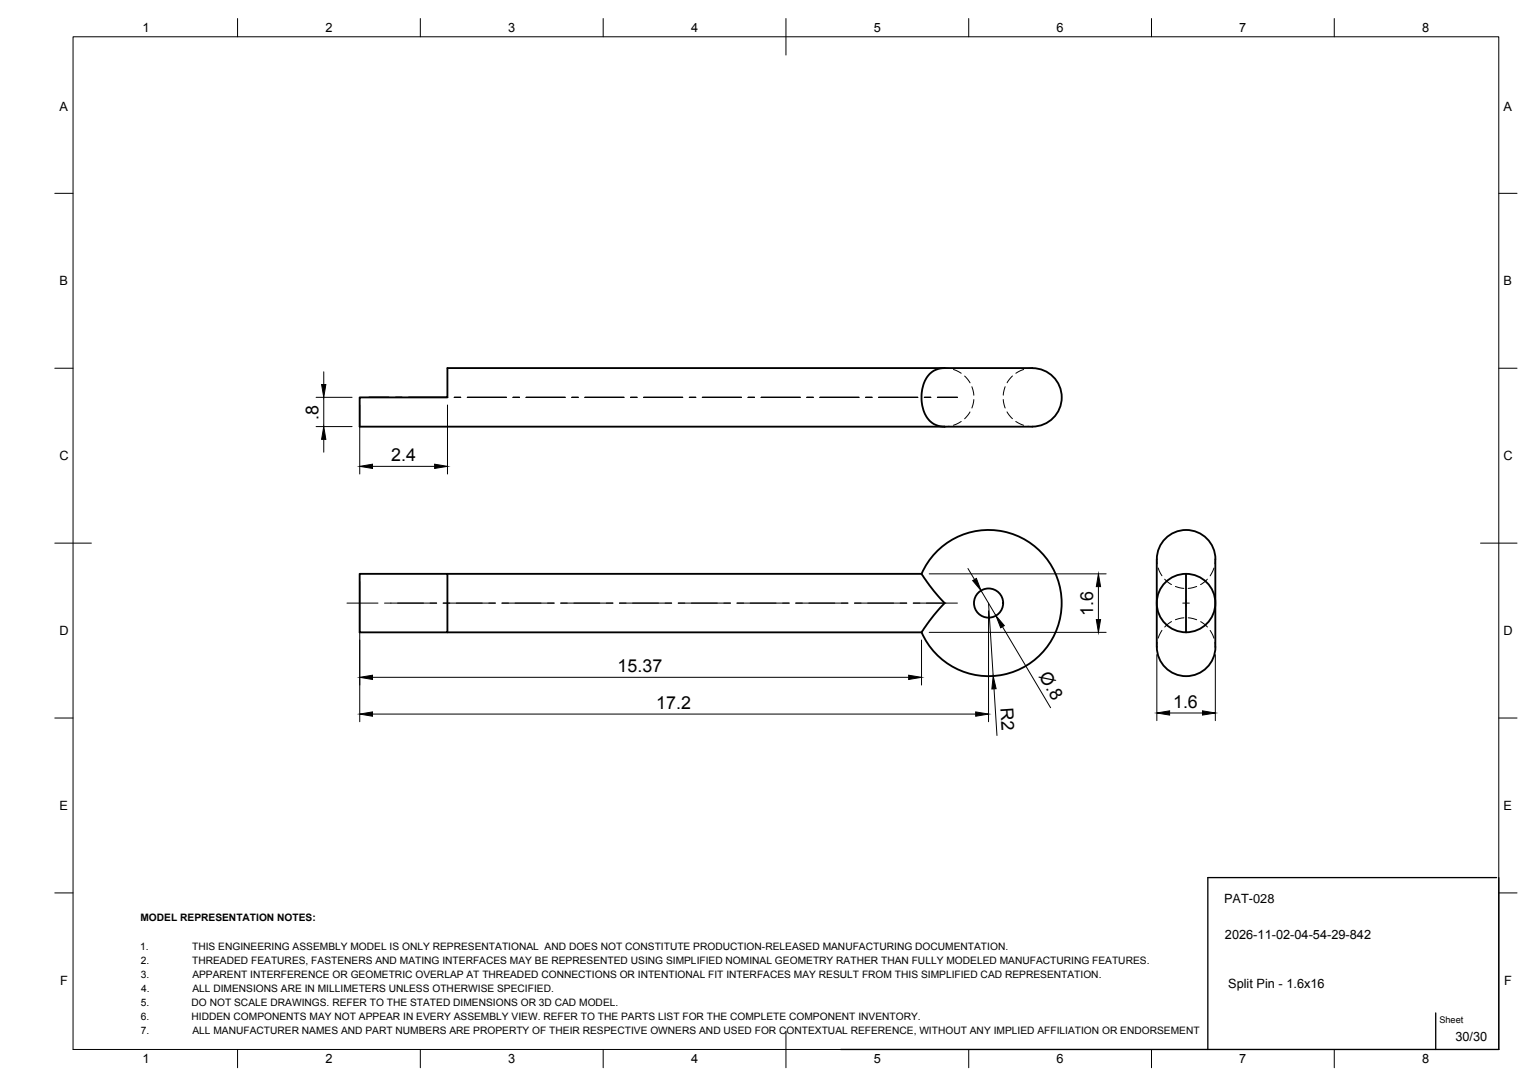
ISO-10303-21;
HEADER;
/* Generated by software containing ST-Developer
 * from STEP Tools, Inc. (www.steptools.com) 
 */

FILE_DESCRIPTION(
/* description */ ('Cylinder foot and clevis mount kit'),
/* implementation_level */ '2;1');

FILE_NAME(
/* name */ 'Split Pin - 1.6x16.step',
/* time_stamp */ '2026-10-27T20:10:43-07:00',
/* author */ (''),
/* organization */ (''),
/* preprocessor_version */ 'ST-DEVELOPER v20.2',
/* originating_system */ 'Autodesk Translation Framework v15.17.0.0',
/* authorisation */ '');

FILE_SCHEMA (('AUTOMOTIVE_DESIGN { 1 0 10303 214 3 1 1 }'));
ENDSEC;

DATA;
#10=MECHANICAL_DESIGN_GEOMETRIC_PRESENTATION_REPRESENTATION('',(#365),#9102);
#17=B_SPLINE_CURVE_WITH_KNOTS('',3,(#8955,#8956,#8957,#8958,#8959,#8960,
#8961,#8962,#8963,#8964,#8965,#8966,#8967,#8968,#8969,#8970,#8971,#8972,
#8973,#8974,#8975,#8976,#8977,#8978,#8979,#8980),.UNSPECIFIED.,.F.,.F.,
(4,2,2,2,2,2,2,2,2,2,2,2,4),(-0.00054581412719389,0.,0.0281583564005144,
0.0618496465371181,0.0905865724114538,0.120694112793616,0.144966158459363,
0.16923820412511,0.199345744507272,0.228082670381608,0.261773960518212,
0.289932316918681,0.290478131045882),.UNSPECIFIED.);
#18=B_SPLINE_CURVE_WITH_KNOTS('',3,(#8981,#8982,#8983,#8984,#8985,#8986,
#8987,#8988,#8989,#8990,#8991,#8992,#8993,#8994,#8995,#8996,#8997,#8998,
#8999,#9000,#9001,#9002,#9003,#9004,#9005,#9006),.UNSPECIFIED.,.F.,.F.,
(4,2,2,2,2,2,2,2,2,2,2,2,4),(-0.000545814127196571,0.,0.0281583564006391,
0.0618496465374156,0.0905865724118984,0.120694112794215,0.144966158460086,
0.169238204125958,0.199345744508275,0.228082670382758,0.261773960519534,
0.289932316920171,0.29047813104737),.UNSPECIFIED.);
#34=TOROIDAL_SURFACE('',#5868,0.12,0.08);
#309=SHAPE_REPRESENTATION_RELATIONSHIP('SRR','None',#9258,#337);
#337=ADVANCED_BREP_SHAPE_REPRESENTATION('',(#391),#9101);
#365=STYLED_ITEM('',(#9460),#391);
#391=MANIFOLD_SOLID_BREP('Body1',#4953);
#494=FACE_BOUND('',#1405,.T.);
#692=PLANE('',#5871);
#693=PLANE('',#5873);
#694=PLANE('',#5877);
#996=FACE_OUTER_BOUND('',#1404,.T.);
#997=FACE_OUTER_BOUND('',#1406,.T.);
#998=FACE_OUTER_BOUND('',#1407,.T.);
#999=FACE_OUTER_BOUND('',#1408,.T.);
#1000=FACE_OUTER_BOUND('',#1409,.T.);
#1404=EDGE_LOOP('',(#4497,#4498,#4499,#4500));
#1405=EDGE_LOOP('',(#4501,#4502));
#1406=EDGE_LOOP('',(#4503,#4504));
#1407=EDGE_LOOP('',(#4505,#4506,#4507,#4508));
#1408=EDGE_LOOP('',(#4509,#4510,#4511,#4512,#4513,#4514,#4515,#4516,#4517));
#1409=EDGE_LOOP('',(#4518,#4519,#4520));
#1754=LINE('',#9011,#2103);
#1755=LINE('',#9014,#2104);
#1756=LINE('',#9016,#2105);
#1757=LINE('',#9017,#2106);
#1758=LINE('',#9021,#2107);
#2103=VECTOR('',#7455,1.);
#2104=VECTOR('',#7458,1.);
#2105=VECTOR('',#7459,1.);
#2106=VECTOR('',#7460,1.);
#2107=VECTOR('',#7465,0.08);
#2323=CIRCLE('',#5869,0.08);
#2324=CIRCLE('',#5870,0.04);
#2325=CIRCLE('',#5872,0.08);
#2326=CIRCLE('',#5875,0.08);
#2327=CIRCLE('',#5876,0.08);
#2704=VERTEX_POINT('',#8950);
#2705=VERTEX_POINT('',#8953);
#2706=VERTEX_POINT('',#8954);
#2707=VERTEX_POINT('',#9008);
#2708=VERTEX_POINT('',#9009);
#2709=VERTEX_POINT('',#9013);
#2710=VERTEX_POINT('',#9015);
#2711=VERTEX_POINT('',#9019);
#3303=EDGE_CURVE('',#2704,#2704,#2323,.T.);
#3304=EDGE_CURVE('',#2704,#2704,#2324,.T.);
#3305=EDGE_CURVE('',#2705,#2706,#17,.T.);
#3306=EDGE_CURVE('',#2706,#2705,#18,.T.);
#3307=EDGE_CURVE('',#2707,#2708,#2325,.T.);
#3308=EDGE_CURVE('',#2707,#2708,#1754,.T.);
#3309=EDGE_CURVE('',#2708,#2709,#1755,.T.);
#3310=EDGE_CURVE('',#2710,#2709,#1756,.T.);
#3311=EDGE_CURVE('',#2707,#2710,#1757,.T.);
#3312=EDGE_CURVE('',#2711,#2710,#2326,.T.);
#3313=EDGE_CURVE('',#2711,#2706,#1758,.T.);
#3314=EDGE_CURVE('',#2709,#2711,#2327,.T.);
#4497=ORIENTED_EDGE('',*,*,#3303,.F.);
#4498=ORIENTED_EDGE('',*,*,#3304,.T.);
#4499=ORIENTED_EDGE('',*,*,#3303,.T.);
#4500=ORIENTED_EDGE('',*,*,#3304,.F.);
#4501=ORIENTED_EDGE('',*,*,#3305,.F.);
#4502=ORIENTED_EDGE('',*,*,#3306,.F.);
#4503=ORIENTED_EDGE('',*,*,#3307,.T.);
#4504=ORIENTED_EDGE('',*,*,#3308,.F.);
#4505=ORIENTED_EDGE('',*,*,#3308,.T.);
#4506=ORIENTED_EDGE('',*,*,#3309,.T.);
#4507=ORIENTED_EDGE('',*,*,#3310,.F.);
#4508=ORIENTED_EDGE('',*,*,#3311,.F.);
#4509=ORIENTED_EDGE('',*,*,#3307,.F.);
#4510=ORIENTED_EDGE('',*,*,#3311,.T.);
#4511=ORIENTED_EDGE('',*,*,#3312,.F.);
#4512=ORIENTED_EDGE('',*,*,#3313,.T.);
#4513=ORIENTED_EDGE('',*,*,#3306,.T.);
#4514=ORIENTED_EDGE('',*,*,#3305,.T.);
#4515=ORIENTED_EDGE('',*,*,#3313,.F.);
#4516=ORIENTED_EDGE('',*,*,#3314,.F.);
#4517=ORIENTED_EDGE('',*,*,#3309,.F.);
#4518=ORIENTED_EDGE('',*,*,#3314,.T.);
#4519=ORIENTED_EDGE('',*,*,#3312,.T.);
#4520=ORIENTED_EDGE('',*,*,#3310,.T.);
#4617=CYLINDRICAL_SURFACE('',#5874,0.08);
#4919=ADVANCED_FACE('',(#996,#494),#34,.T.);
#4920=ADVANCED_FACE('',(#997),#692,.F.);
#4921=ADVANCED_FACE('',(#998),#693,.T.);
#4922=ADVANCED_FACE('',(#999),#4617,.T.);
#4923=ADVANCED_FACE('',(#1000),#694,.F.);
#4953=CLOSED_SHELL('',(#4919,#4920,#4921,#4922,#4923));
#5867=AXIS2_PLACEMENT_3D('',#8948,#7443,#7444);
#5868=AXIS2_PLACEMENT_3D('',#8949,#7445,#7446);
#5869=AXIS2_PLACEMENT_3D('',#8951,#7447,#7448);
#5870=AXIS2_PLACEMENT_3D('',#8952,#7449,#7450);
#5871=AXIS2_PLACEMENT_3D('',#9007,#7451,#7452);
#5872=AXIS2_PLACEMENT_3D('',#9010,#7453,#7454);
#5873=AXIS2_PLACEMENT_3D('',#9012,#7456,#7457);
#5874=AXIS2_PLACEMENT_3D('',#9018,#7461,#7462);
#5875=AXIS2_PLACEMENT_3D('',#9020,#7463,#7464);
#5876=AXIS2_PLACEMENT_3D('',#9022,#7466,#7467);
#5877=AXIS2_PLACEMENT_3D('',#9023,#7468,#7469);
#7443=DIRECTION('axis',(0.,0.,1.));
#7444=DIRECTION('refdir',(1.,0.,0.));
#7445=DIRECTION('center_axis',(-1.,0.,0.));
#7446=DIRECTION('ref_axis',(0.,0.,1.));
#7447=DIRECTION('center_axis',(0.,-1.,1.38777878078145E-16));
#7448=DIRECTION('ref_axis',(0.,-1.38777878078145E-16,-1.));
#7449=DIRECTION('center_axis',(1.,0.,0.));
#7450=DIRECTION('ref_axis',(0.,0.,1.));
#7451=DIRECTION('center_axis',(0.,1.,0.));
#7452=DIRECTION('ref_axis',(1.,0.,0.));
#7453=DIRECTION('center_axis',(0.,-1.,0.));
#7454=DIRECTION('ref_axis',(1.,0.,0.));
#7455=DIRECTION('',(0.,0.,1.));
#7456=DIRECTION('center_axis',(1.,0.,0.));
#7457=DIRECTION('ref_axis',(0.,0.,1.));
#7458=DIRECTION('',(0.,-1.,0.));
#7459=DIRECTION('',(0.,0.,1.));
#7460=DIRECTION('',(0.,-1.,0.));
#7461=DIRECTION('center_axis',(0.,-1.,0.));
#7462=DIRECTION('ref_axis',(1.,0.,0.));
#7463=DIRECTION('center_axis',(0.,-1.,0.));
#7464=DIRECTION('ref_axis',(1.,0.,0.));
#7465=DIRECTION('',(0.,1.,0.));
#7466=DIRECTION('center_axis',(0.,-1.,0.));
#7467=DIRECTION('ref_axis',(1.,0.,0.));
#7468=DIRECTION('center_axis',(0.,1.,0.));
#7469=DIRECTION('ref_axis',(1.,0.,0.));
#8948=CARTESIAN_POINT('',(0.,0.,0.));
#8949=CARTESIAN_POINT('Origin',(0.,0.12,0.));
#8950=CARTESIAN_POINT('',(-9.79717439317883E-18,0.12,-0.04));
#8951=CARTESIAN_POINT('Origin',(0.,0.12,-0.12));
#8952=CARTESIAN_POINT('Origin',(9.79717439317883E-18,0.12,0.));
#8953=CARTESIAN_POINT('',(0.08,-4.89858719658941E-18,7.34788079488412E-18));
#8954=CARTESIAN_POINT('',(-0.08,-4.89858719658941E-18,7.34788079488412E-18));
#8955=CARTESIAN_POINT('Ctrl Pts',(0.08,-4.89858719658941E-18,7.34788079488412E-18));
#8956=CARTESIAN_POINT('Ctrl Pts',(0.08,-0.00012864962353541,0.000128649623535413));
#8957=CARTESIAN_POINT('Ctrl Pts',(0.0799996896739287,-0.00025719571182076,
0.000257402596003253));
#8958=CARTESIAN_POINT('Ctrl Pts',(0.0799669711262291,-0.00701193164572964,
0.00703384588894362));
#8959=CARTESIAN_POINT('Ctrl Pts',(0.0791054994909294,-0.0133457972655825,
0.0139383126556792));
#8960=CARTESIAN_POINT('Ctrl Pts',(0.0749700088488058,-0.0265076530862524,
0.0292212026164895));
#8961=CARTESIAN_POINT('Ctrl Pts',(0.0712702072865517,-0.0331317062461458,
0.0375603420117568));
#8962=CARTESIAN_POINT('Ctrl Pts',(0.0612858949407667,-0.0440683985740427,
0.0520545604187517));
#8963=CARTESIAN_POINT('Ctrl Pts',(0.0555090276731744,-0.0485199197794574,
0.0582717815295611));
#8964=CARTESIAN_POINT('Ctrl Pts',(0.0412398082144208,-0.0561090538733877,
0.0691638397919718));
#8965=CARTESIAN_POINT('Ctrl Pts',(0.0327878980890048,-0.059089642483296,
0.0736229049587921));
#8966=CARTESIAN_POINT('Ctrl Pts',(0.0159233027310102,-0.0625179833270725,
0.0787936360751706));
#8967=CARTESIAN_POINT('Ctrl Pts',(0.00801661414593076,-0.0633030277982336,
0.08));
#8968=CARTESIAN_POINT('Ctrl Pts',(-0.00801661414593074,-0.0633030277982336,
0.08));
#8969=CARTESIAN_POINT('Ctrl Pts',(-0.0159233027310102,-0.0625179833270726,
0.0787936360751706));
#8970=CARTESIAN_POINT('Ctrl Pts',(-0.0327878980890049,-0.059089642483296,
0.0736229049587921));
#8971=CARTESIAN_POINT('Ctrl Pts',(-0.0412398082144209,-0.0561090538733877,
0.0691638397919717));
#8972=CARTESIAN_POINT('Ctrl Pts',(-0.0555090276731744,-0.0485199197794574,
0.0582717815295611));
#8973=CARTESIAN_POINT('Ctrl Pts',(-0.0612858949407667,-0.0440683985740427,
0.0520545604187517));
#8974=CARTESIAN_POINT('Ctrl Pts',(-0.0712702072865517,-0.0331317062461458,
0.0375603420117568));
#8975=CARTESIAN_POINT('Ctrl Pts',(-0.0749700088488058,-0.0265076530862524,
0.0292212026164895));
#8976=CARTESIAN_POINT('Ctrl Pts',(-0.0791054994909264,-0.0133457972655921,
0.0139383126556903));
#8977=CARTESIAN_POINT('Ctrl Pts',(-0.0799669711262287,-0.00701193164579759,
0.0070338458890125));
#8978=CARTESIAN_POINT('Ctrl Pts',(-0.0799996896739287,-0.000257195711817665,
0.000257402596000083));
#8979=CARTESIAN_POINT('Ctrl Pts',(-0.08,-0.000128649623538514,0.000128649623538516));
#8980=CARTESIAN_POINT('Ctrl Pts',(-0.08,-4.89858719658941E-18,7.34788079488412E-18));
#8981=CARTESIAN_POINT('Ctrl Pts',(-0.08,-4.89858719658941E-18,7.34788079488412E-18));
#8982=CARTESIAN_POINT('Ctrl Pts',(-0.08,-0.000128649623536042,-0.00012864962353603));
#8983=CARTESIAN_POINT('Ctrl Pts',(-0.0799996896739287,-0.000257195711820127,
-0.000257402596002604));
#8984=CARTESIAN_POINT('Ctrl Pts',(-0.0799669711262289,-0.0070119316457589,
-0.00703384588897312));
#8985=CARTESIAN_POINT('Ctrl Pts',(-0.0791054994909281,-0.0133457972655867,
-0.0139383126556841));
#8986=CARTESIAN_POINT('Ctrl Pts',(-0.0749700088488058,-0.0265076530862525,
-0.0292212026164896));
#8987=CARTESIAN_POINT('Ctrl Pts',(-0.0712702072865516,-0.0331317062461459,
-0.0375603420117568));
#8988=CARTESIAN_POINT('Ctrl Pts',(-0.0612858949407667,-0.0440683985740427,
-0.0520545604187517));
#8989=CARTESIAN_POINT('Ctrl Pts',(-0.0555090276731744,-0.0485199197794574,
-0.0582717815295611));
#8990=CARTESIAN_POINT('Ctrl Pts',(-0.0412398082144209,-0.0561090538733877,
-0.0691638397919717));
#8991=CARTESIAN_POINT('Ctrl Pts',(-0.0327878980890049,-0.059089642483296,
-0.0736229049587921));
#8992=CARTESIAN_POINT('Ctrl Pts',(-0.0159233027310101,-0.0625179833270725,
-0.0787936360751706));
#8993=CARTESIAN_POINT('Ctrl Pts',(-0.00801661414593069,-0.0633030277982336,
-0.08));
#8994=CARTESIAN_POINT('Ctrl Pts',(0.0080166141459307,-0.0633030277982336,
-0.08));
#8995=CARTESIAN_POINT('Ctrl Pts',(0.0159233027310101,-0.0625179833270725,
-0.0787936360751706));
#8996=CARTESIAN_POINT('Ctrl Pts',(0.0327878980890049,-0.0590896424832959,
-0.0736229049587921));
#8997=CARTESIAN_POINT('Ctrl Pts',(0.0412398082144209,-0.0561090538733877,
-0.0691638397919717));
#8998=CARTESIAN_POINT('Ctrl Pts',(0.0555090276731744,-0.0485199197794574,
-0.0582717815295611));
#8999=CARTESIAN_POINT('Ctrl Pts',(0.0612858949407666,-0.0440683985740428,
-0.0520545604187518));
#9000=CARTESIAN_POINT('Ctrl Pts',(0.0712702072865517,-0.0331317062461458,
-0.0375603420117568));
#9001=CARTESIAN_POINT('Ctrl Pts',(0.0749700088488058,-0.0265076530862524,
-0.0292212026164895));
#9002=CARTESIAN_POINT('Ctrl Pts',(0.079105499490928,-0.013345797265587,
-0.0139383126556845));
#9003=CARTESIAN_POINT('Ctrl Pts',(0.0799669711262289,-0.00701193164576148,
-0.00703384588897579));
#9004=CARTESIAN_POINT('Ctrl Pts',(0.0799996896739287,-0.000257195711819584,
-0.000257402596002039));
#9005=CARTESIAN_POINT('Ctrl Pts',(0.08,-0.000128649623536605,-0.000128649623536593));
#9006=CARTESIAN_POINT('Ctrl Pts',(0.08,-4.89858719658941E-18,7.34788079488412E-18));
#9007=CARTESIAN_POINT('Origin',(0.04,-1.36,0.));
#9008=CARTESIAN_POINT('',(0.,-1.36,-0.08));
#9009=CARTESIAN_POINT('',(0.,-1.36,0.08));
#9010=CARTESIAN_POINT('Origin',(0.,-1.36,0.));
#9011=CARTESIAN_POINT('',(0.,-1.36,-0.04));
#9012=CARTESIAN_POINT('Origin',(0.,0.,-0.08));
#9013=CARTESIAN_POINT('',(0.,-1.6,0.08));
#9014=CARTESIAN_POINT('',(0.,0.,0.08));
#9015=CARTESIAN_POINT('',(0.,-1.6,-0.08));
#9016=CARTESIAN_POINT('',(0.,-1.6,-0.09));
#9017=CARTESIAN_POINT('',(0.,0.,-0.08));
#9018=CARTESIAN_POINT('Origin',(0.,0.,0.));
#9019=CARTESIAN_POINT('',(-0.08,-1.6,-9.79717439317883E-18));
#9020=CARTESIAN_POINT('Origin',(0.,-1.6,0.));
#9021=CARTESIAN_POINT('',(-0.08,0.,-9.79717439317883E-18));
#9022=CARTESIAN_POINT('Origin',(0.,-1.6,0.));
#9023=CARTESIAN_POINT('Origin',(-0.04,-1.6,0.));
#9068=UNCERTAINTY_MEASURE_WITH_UNIT(LENGTH_MEASURE(0.001),#9103,
'DISTANCE_ACCURACY_VALUE',
'Maximum model space distance between geometric entities at asserted c
onnectivities');
#9069=UNCERTAINTY_MEASURE_WITH_UNIT(LENGTH_MEASURE(0.001),#9103,
'DISTANCE_ACCURACY_VALUE',
'Maximum model space distance between geometric entities at asserted c
onnectivities');
#9101=(
GEOMETRIC_REPRESENTATION_CONTEXT(3)
GLOBAL_UNCERTAINTY_ASSIGNED_CONTEXT((#9068))
GLOBAL_UNIT_ASSIGNED_CONTEXT((#9103,#9105,#9106))
REPRESENTATION_CONTEXT('','3D')
);
#9102=(
GEOMETRIC_REPRESENTATION_CONTEXT(3)
GLOBAL_UNCERTAINTY_ASSIGNED_CONTEXT((#9069))
GLOBAL_UNIT_ASSIGNED_CONTEXT((#9103,#9105,#9106))
REPRESENTATION_CONTEXT('','3D')
);
#9103=(
LENGTH_UNIT()
NAMED_UNIT(*)
SI_UNIT(.CENTI.,.METRE.)
);
#9105=(
NAMED_UNIT(*)
PLANE_ANGLE_UNIT()
SI_UNIT($,.RADIAN.)
);
#9106=(
NAMED_UNIT(*)
SI_UNIT($,.STERADIAN.)
SOLID_ANGLE_UNIT()
);
#9138=SHAPE_DEFINITION_REPRESENTATION(#9213,#9258);
#9213=PRODUCT_DEFINITION_SHAPE('',$,#9291);
#9258=SHAPE_REPRESENTATION('',(#5867),#9101);
#9259=PRODUCT_DEFINITION_CONTEXT('part definition',#9357,'design');
#9291=PRODUCT_DEFINITION('Split Pin - 1.6x16','Split Pin - 1.6x16',#9323,
#9259);
#9323=PRODUCT_DEFINITION_FORMATION('',$,#9390);
#9357=APPLICATION_CONTEXT(
'Core Data for Automotive Mechanical Design Process');
#9358=PRODUCT_CONTEXT('part definition',#9357,'mechanical');
#9390=PRODUCT('Split Pin - 1.6x16','Split Pin - 1.6x16',
'Split Pin - 1.6x16',(#9358));
#9454=COLOUR_RGB('Grey',0.48,0.52,0.57);
#9455=FILL_AREA_STYLE_COLOUR('',#9454);
#9456=FILL_AREA_STYLE('',(#9455));
#9457=SURFACE_STYLE_FILL_AREA(#9456);
#9458=SURFACE_SIDE_STYLE('',(#9457));
#9459=SURFACE_STYLE_USAGE(.BOTH.,#9458);
#9460=PRESENTATION_STYLE_ASSIGNMENT((#9459));
ENDSEC;
END-ISO-10303-21;
